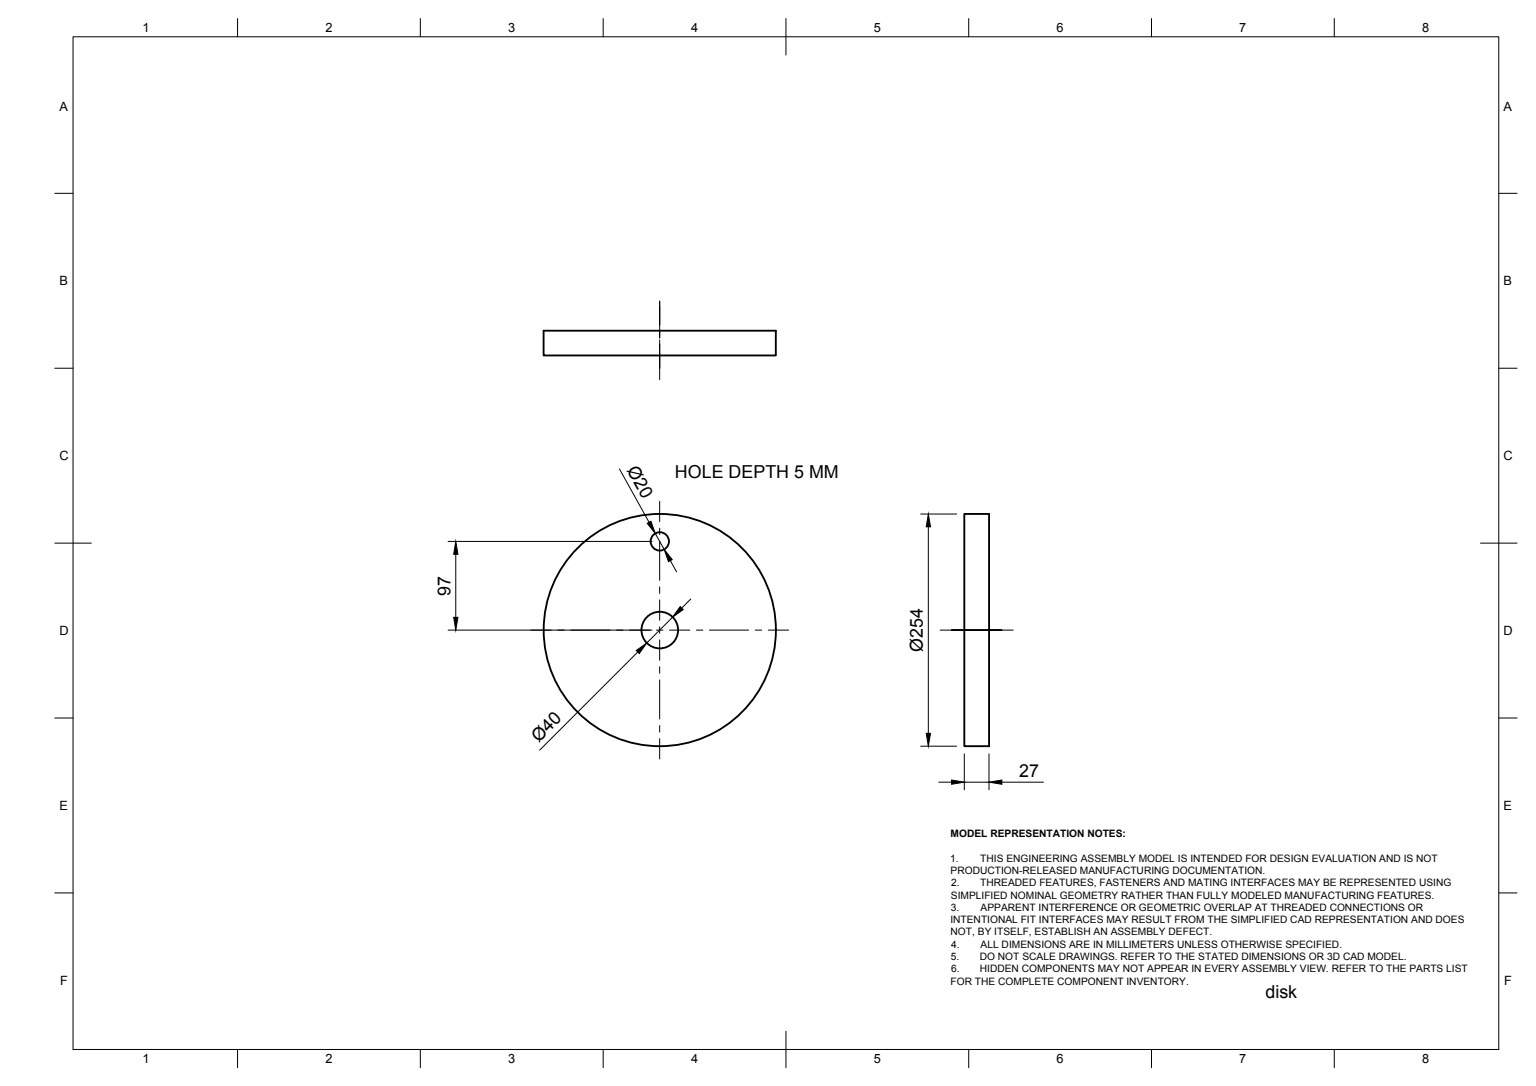
ISO-10303-21;
HEADER;
/* Generated by software containing ST-Developer
 * from STEP Tools, Inc. (www.steptools.com) 
 */

FILE_DESCRIPTION(
/* description */ (''),
/* implementation_level */ '2;1');

FILE_NAME(
/* name */ 'Disk.step',
/* time_stamp */ '2026-10-05T19:45:59-07:00',
/* author */ (''),
/* organization */ (''),
/* preprocessor_version */ 'ST-DEVELOPER v20.2',
/* originating_system */ 'Autodesk Translation Framework v15.15.0.0',
/* authorisation */ '');

FILE_SCHEMA (('AUTOMOTIVE_DESIGN { 1 0 10303 214 3 1 1 }'));
ENDSEC;

DATA;
#10=MECHANICAL_DESIGN_GEOMETRIC_PRESENTATION_REPRESENTATION('',(#92),#2462);
#57=FACE_BOUND('',#263,.T.);
#58=FACE_BOUND('',#264,.T.);
#74=SHAPE_REPRESENTATION_RELATIONSHIP('SRR','None',#2500,#83);
#83=ADVANCED_BREP_SHAPE_REPRESENTATION('',(#101),#2455);
#92=STYLED_ITEM('',(#2553),#101);
#101=MANIFOLD_SOLID_BREP('Body1',#1329);
#118=PLANE('',#1468);
#119=PLANE('',#1469);
#120=PLANE('',#1474);
#121=PLANE('',#1477);
#180=FACE_OUTER_BOUND('',#260,.T.);
#181=FACE_OUTER_BOUND('',#261,.T.);
#182=FACE_OUTER_BOUND('',#262,.T.);
#183=FACE_OUTER_BOUND('',#265,.T.);
#184=FACE_OUTER_BOUND('',#266,.T.);
#185=FACE_OUTER_BOUND('',#267,.T.);
#186=FACE_OUTER_BOUND('',#268,.T.);
#260=EDGE_LOOP('',(#960,#961,#962,#963));
#261=EDGE_LOOP('',(#964));
#262=EDGE_LOOP('',(#965));
#263=EDGE_LOOP('',(#966));
#264=EDGE_LOOP('',(#967));
#265=EDGE_LOOP('',(#968,#969,#970,#971));
#266=EDGE_LOOP('',(#972));
#267=EDGE_LOOP('',(#973,#974,#975,#976));
#268=EDGE_LOOP('',(#977));
#363=LINE('',#2062,#482);
#364=LINE('',#2072,#483);
#365=LINE('',#2077,#484);
#482=VECTOR('',#1664,10.);
#483=VECTOR('',#1677,20.);
#484=VECTOR('',#1684,127.);
#588=CIRCLE('',#1466,10.);
#589=CIRCLE('',#1467,10.);
#590=CIRCLE('',#1470,127.);
#591=CIRCLE('',#1471,20.);
#592=CIRCLE('',#1473,20.);
#593=CIRCLE('',#1476,127.);
#643=VERTEX_POINT('',#2059);
#644=VERTEX_POINT('',#2061);
#645=VERTEX_POINT('',#2066);
#646=VERTEX_POINT('',#2068);
#647=VERTEX_POINT('',#2071);
#648=VERTEX_POINT('',#2076);
#761=EDGE_CURVE('',#643,#643,#588,.T.);
#762=EDGE_CURVE('',#643,#644,#363,.T.);
#763=EDGE_CURVE('',#644,#644,#589,.T.);
#764=EDGE_CURVE('',#645,#645,#590,.T.);
#765=EDGE_CURVE('',#646,#646,#591,.T.);
#766=EDGE_CURVE('',#646,#647,#364,.T.);
#767=EDGE_CURVE('',#647,#647,#592,.T.);
#768=EDGE_CURVE('',#645,#648,#365,.T.);
#769=EDGE_CURVE('',#648,#648,#593,.F.);
#960=ORIENTED_EDGE('',*,*,#761,.F.);
#961=ORIENTED_EDGE('',*,*,#762,.T.);
#962=ORIENTED_EDGE('',*,*,#763,.T.);
#963=ORIENTED_EDGE('',*,*,#762,.F.);
#964=ORIENTED_EDGE('',*,*,#763,.F.);
#965=ORIENTED_EDGE('',*,*,#764,.T.);
#966=ORIENTED_EDGE('',*,*,#761,.T.);
#967=ORIENTED_EDGE('',*,*,#765,.T.);
#968=ORIENTED_EDGE('',*,*,#765,.F.);
#969=ORIENTED_EDGE('',*,*,#766,.T.);
#970=ORIENTED_EDGE('',*,*,#767,.T.);
#971=ORIENTED_EDGE('',*,*,#766,.F.);
#972=ORIENTED_EDGE('',*,*,#767,.F.);
#973=ORIENTED_EDGE('',*,*,#764,.F.);
#974=ORIENTED_EDGE('',*,*,#768,.T.);
#975=ORIENTED_EDGE('',*,*,#769,.F.);
#976=ORIENTED_EDGE('',*,*,#768,.F.);
#977=ORIENTED_EDGE('',*,*,#769,.T.);
#1231=CYLINDRICAL_SURFACE('',#1465,10.);
#1232=CYLINDRICAL_SURFACE('',#1472,20.);
#1233=CYLINDRICAL_SURFACE('',#1475,127.);
#1262=ADVANCED_FACE('',(#180),#1231,.F.);
#1263=ADVANCED_FACE('',(#181),#118,.T.);
#1264=ADVANCED_FACE('',(#182,#57,#58),#119,.F.);
#1265=ADVANCED_FACE('',(#183),#1232,.F.);
#1266=ADVANCED_FACE('',(#184),#120,.T.);
#1267=ADVANCED_FACE('',(#185),#1233,.T.);
#1268=ADVANCED_FACE('',(#186),#121,.T.);
#1329=CLOSED_SHELL('',(#1262,#1263,#1264,#1265,#1266,#1267,#1268));
#1464=AXIS2_PLACEMENT_3D('',#2057,#1658,#1659);
#1465=AXIS2_PLACEMENT_3D('',#2058,#1660,#1661);
#1466=AXIS2_PLACEMENT_3D('',#2060,#1662,#1663);
#1467=AXIS2_PLACEMENT_3D('',#2063,#1665,#1666);
#1468=AXIS2_PLACEMENT_3D('',#2064,#1667,#1668);
#1469=AXIS2_PLACEMENT_3D('',#2065,#1669,#1670);
#1470=AXIS2_PLACEMENT_3D('',#2067,#1671,#1672);
#1471=AXIS2_PLACEMENT_3D('',#2069,#1673,#1674);
#1472=AXIS2_PLACEMENT_3D('',#2070,#1675,#1676);
#1473=AXIS2_PLACEMENT_3D('',#2073,#1678,#1679);
#1474=AXIS2_PLACEMENT_3D('',#2074,#1680,#1681);
#1475=AXIS2_PLACEMENT_3D('',#2075,#1682,#1683);
#1476=AXIS2_PLACEMENT_3D('',#2078,#1685,#1686);
#1477=AXIS2_PLACEMENT_3D('',#2079,#1687,#1688);
#1658=DIRECTION('axis',(0.,0.,1.));
#1659=DIRECTION('refdir',(1.,0.,0.));
#1660=DIRECTION('center_axis',(0.,0.,-1.));
#1661=DIRECTION('ref_axis',(-1.,0.,0.));
#1662=DIRECTION('center_axis',(0.,0.,-1.));
#1663=DIRECTION('ref_axis',(-1.,0.,0.));
#1664=DIRECTION('',(0.,0.,-1.));
#1665=DIRECTION('center_axis',(0.,0.,-1.));
#1666=DIRECTION('ref_axis',(-1.,0.,0.));
#1667=DIRECTION('center_axis',(0.,0.,1.));
#1668=DIRECTION('ref_axis',(-1.,0.,0.));
#1669=DIRECTION('center_axis',(0.,0.,-1.));
#1670=DIRECTION('ref_axis',(-1.,0.,0.));
#1671=DIRECTION('center_axis',(0.,0.,1.));
#1672=DIRECTION('ref_axis',(-1.,0.,0.));
#1673=DIRECTION('center_axis',(0.,0.,-1.));
#1674=DIRECTION('ref_axis',(-1.,0.,0.));
#1675=DIRECTION('center_axis',(0.,0.,-1.));
#1676=DIRECTION('ref_axis',(-1.,0.,0.));
#1677=DIRECTION('',(0.,0.,-1.));
#1678=DIRECTION('center_axis',(0.,0.,-1.));
#1679=DIRECTION('ref_axis',(-1.,0.,0.));
#1680=DIRECTION('center_axis',(0.,0.,1.));
#1681=DIRECTION('ref_axis',(-1.,0.,0.));
#1682=DIRECTION('center_axis',(0.,0.,1.));
#1683=DIRECTION('ref_axis',(-1.,0.,0.));
#1684=DIRECTION('',(0.,0.,-1.));
#1685=DIRECTION('center_axis',(0.,0.,1.));
#1686=DIRECTION('ref_axis',(-1.,0.,0.));
#1687=DIRECTION('center_axis',(0.,0.,-1.));
#1688=DIRECTION('ref_axis',(-1.,0.,0.));
#2057=CARTESIAN_POINT('',(0.,0.,0.));
#2058=CARTESIAN_POINT('Origin',(-205.724822686805,97.,19.9999999999958));
#2059=CARTESIAN_POINT('',(-195.724822686805,97.,14.9999999999958));
#2060=CARTESIAN_POINT('Origin',(-205.724822686805,97.,14.9999999999958));
#2061=CARTESIAN_POINT('',(-195.724822686805,97.,9.9999999999958));
#2062=CARTESIAN_POINT('',(-195.724822686805,97.,19.9999999999958));
#2063=CARTESIAN_POINT('Origin',(-205.724822686805,97.,9.9999999999958));
#2064=CARTESIAN_POINT('Origin',(-205.724822686805,97.,9.9999999999958));
#2065=CARTESIAN_POINT('Origin',(-205.724822686805,0.,14.9999999999958));
#2066=CARTESIAN_POINT('',(-78.724822686805,1.55530143491714E-14,14.9999999999958));
#2067=CARTESIAN_POINT('Origin',(-205.724822686805,0.,14.9999999999958));
#2068=CARTESIAN_POINT('',(-185.724822686805,-2.44929359829471E-15,14.9999999999958));
#2069=CARTESIAN_POINT('Origin',(-205.724822686805,0.,14.9999999999958));
#2070=CARTESIAN_POINT('Origin',(-205.724822686805,0.,0.));
#2071=CARTESIAN_POINT('',(-185.724822686805,2.44929359829471E-15,-10.));
#2072=CARTESIAN_POINT('',(-185.724822686805,-2.44929359829471E-15,0.));
#2073=CARTESIAN_POINT('Origin',(-205.724822686805,0.,-10.));
#2074=CARTESIAN_POINT('Origin',(-205.724822686805,0.,-10.));
#2075=CARTESIAN_POINT('Origin',(-205.724822686805,0.,-20.));
#2076=CARTESIAN_POINT('',(-78.7248226868051,1.55530143491714E-14,-12.));
#2077=CARTESIAN_POINT('',(-78.724822686805,1.55530143491714E-14,-20.));
#2078=CARTESIAN_POINT('Origin',(-205.724822686805,0.,-12.));
#2079=CARTESIAN_POINT('Origin',(-205.724822686805,0.,-12.));
#2444=UNCERTAINTY_MEASURE_WITH_UNIT(LENGTH_MEASURE(0.01),#2463,
'DISTANCE_ACCURACY_VALUE',
'Maximum model space distance between geometric entities at asserted c
onnectivities');
#2451=UNCERTAINTY_MEASURE_WITH_UNIT(LENGTH_MEASURE(0.01),#2463,
'DISTANCE_ACCURACY_VALUE',
'Maximum model space distance between geometric entities at asserted c
onnectivities');
#2455=(
GEOMETRIC_REPRESENTATION_CONTEXT(3)
GLOBAL_UNCERTAINTY_ASSIGNED_CONTEXT((#2444))
GLOBAL_UNIT_ASSIGNED_CONTEXT((#2463,#2465,#2466))
REPRESENTATION_CONTEXT('','3D')
);
#2462=(
GEOMETRIC_REPRESENTATION_CONTEXT(3)
GLOBAL_UNCERTAINTY_ASSIGNED_CONTEXT((#2451))
GLOBAL_UNIT_ASSIGNED_CONTEXT((#2463,#2465,#2466))
REPRESENTATION_CONTEXT('','3D')
);
#2463=(
LENGTH_UNIT()
NAMED_UNIT(*)
SI_UNIT(.MILLI.,.METRE.)
);
#2465=(
NAMED_UNIT(*)
PLANE_ANGLE_UNIT()
SI_UNIT($,.RADIAN.)
);
#2466=(
NAMED_UNIT(*)
SI_UNIT($,.STERADIAN.)
SOLID_ANGLE_UNIT()
);
#2470=SHAPE_DEFINITION_REPRESENTATION(#2480,#2500);
#2480=PRODUCT_DEFINITION_SHAPE('',$,#2511);
#2500=SHAPE_REPRESENTATION('',(#1464),#2455);
#2507=PRODUCT_DEFINITION_CONTEXT('part definition',#2539,'design');
#2511=PRODUCT_DEFINITION('Disk','Disk',#2521,#2507);
#2521=PRODUCT_DEFINITION_FORMATION('',$,#2544);
#2539=APPLICATION_CONTEXT(
'Core Data for Automotive Mechanical Design Process');
#2540=PRODUCT_CONTEXT('part definition',#2539,'mechanical');
#2544=PRODUCT('Disk','Disk',$,(#2540));
#2553=PRESENTATION_STYLE_ASSIGNMENT((#2556));
#2556=SURFACE_STYLE_USAGE(.BOTH.,#2559);
#2559=SURFACE_SIDE_STYLE('',(#2562));
#2562=SURFACE_STYLE_FILL_AREA(#2565);
#2565=FILL_AREA_STYLE('Opaque(179,179,179)',(#2568));
#2568=FILL_AREA_STYLE_COLOUR('Opaque(179,179,179)',#2571);
#2571=COLOUR_RGB('Opaque(179,179,179)', 0.31764706, 0.68627451, 0.89019608);
ENDSEC;
END-ISO-10303-21;
